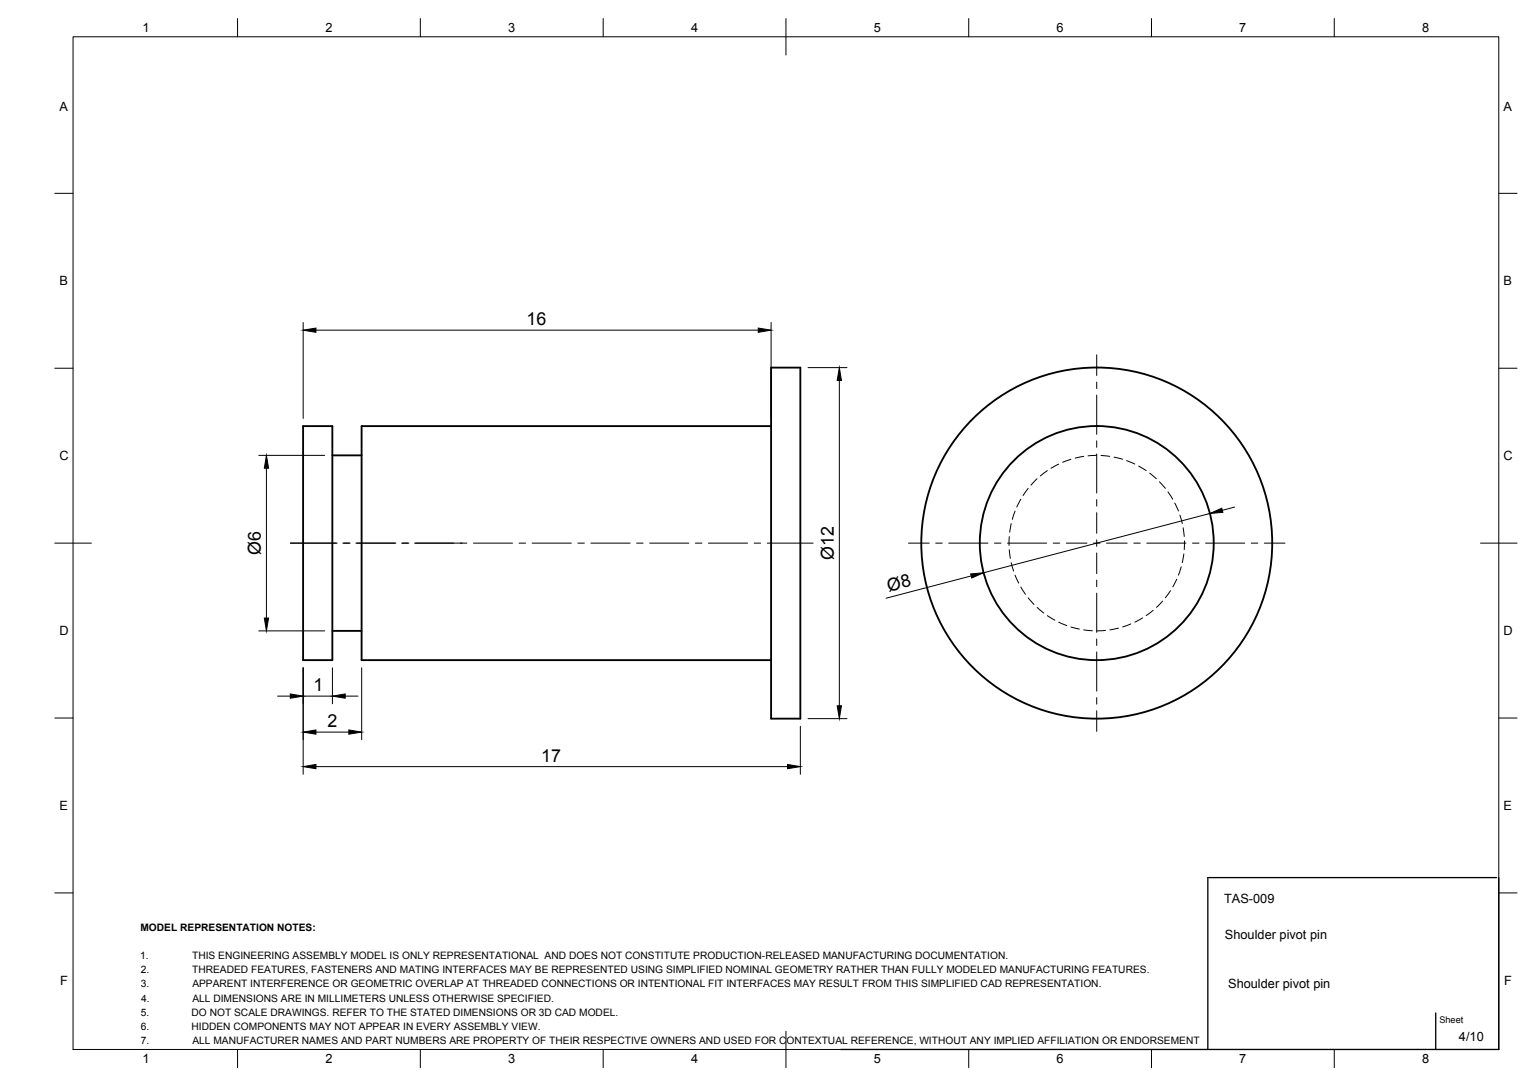
ISO-10303-21;
HEADER;
/* Generated by software containing ST-Developer
 * from STEP Tools, Inc. (www.steptools.com) 
 */

FILE_DESCRIPTION(
/* description */ (''),
/* implementation_level */ '2;1');

FILE_NAME(
/* name */ 'Shoulder pivot pin.step',
/* time_stamp */ '2026-11-12T00:53:40-08:00',
/* author */ (''),
/* organization */ (''),
/* preprocessor_version */ 'ST-DEVELOPER v20.2',
/* originating_system */ 'Autodesk Translation Framework v15.17.0.0',
/* authorisation */ '');

FILE_SCHEMA (('AUTOMOTIVE_DESIGN { 1 0 10303 214 3 1 1 }'));
ENDSEC;

DATA;
#10=MECHANICAL_DESIGN_GEOMETRIC_PRESENTATION_REPRESENTATION('',(#573),#22129);
#555=SHAPE_REPRESENTATION_RELATIONSHIP('SRR','None',#22174,#564);
#564=ADVANCED_BREP_SHAPE_REPRESENTATION('',(#582),#22120);
#573=STYLED_ITEM('',(#22233),#582);
#582=MANIFOLD_SOLID_BREP('Body1',#8804);
#596=FACE_BOUND('',#1528,.T.);
#597=FACE_BOUND('',#1530,.T.);
#598=FACE_BOUND('',#1533,.T.);
#780=PLANE('',#9062);
#781=PLANE('',#9064);
#782=PLANE('',#9068);
#783=PLANE('',#9073);
#784=PLANE('',#9075);
#1037=FACE_OUTER_BOUND('',#1526,.T.);
#1038=FACE_OUTER_BOUND('',#1527,.T.);
#1039=FACE_OUTER_BOUND('',#1529,.T.);
#1040=FACE_OUTER_BOUND('',#1531,.T.);
#1041=FACE_OUTER_BOUND('',#1532,.T.);
#1042=FACE_OUTER_BOUND('',#1534,.T.);
#1043=FACE_OUTER_BOUND('',#1535,.T.);
#1044=FACE_OUTER_BOUND('',#1536,.T.);
#1045=FACE_OUTER_BOUND('',#1537,.T.);
#1526=EDGE_LOOP('',(#6438,#6439,#6440,#6441));
#1527=EDGE_LOOP('',(#6442));
#1528=EDGE_LOOP('',(#6443));
#1529=EDGE_LOOP('',(#6444));
#1530=EDGE_LOOP('',(#6445));
#1531=EDGE_LOOP('',(#6446,#6447,#6448,#6449));
#1532=EDGE_LOOP('',(#6450));
#1533=EDGE_LOOP('',(#6451));
#1534=EDGE_LOOP('',(#6452,#6453,#6454,#6455));
#1535=EDGE_LOOP('',(#6456));
#1536=EDGE_LOOP('',(#6457,#6458,#6459,#6460));
#1537=EDGE_LOOP('',(#6461));
#2316=LINE('',#12207,#3046);
#2317=LINE('',#12218,#3047);
#2318=LINE('',#12226,#3048);
#2319=LINE('',#12230,#3049);
#3046=VECTOR('',#10184,0.3);
#3047=VECTOR('',#10199,0.4);
#3048=VECTOR('',#10208,0.6);
#3049=VECTOR('',#10215,0.4);
#3400=CIRCLE('',#9060,0.3);
#3401=CIRCLE('',#9061,0.3);
#3402=CIRCLE('',#9063,0.4);
#3403=CIRCLE('',#9065,0.4);
#3404=CIRCLE('',#9067,0.4);
#3405=CIRCLE('',#9069,0.6);
#3406=CIRCLE('',#9070,0.4);
#3407=CIRCLE('',#9072,0.6);
#3812=VERTEX_POINT('',#12204);
#3813=VERTEX_POINT('',#12206);
#3814=VERTEX_POINT('',#12210);
#3815=VERTEX_POINT('',#12213);
#3816=VERTEX_POINT('',#12216);
#3817=VERTEX_POINT('',#12220);
#3818=VERTEX_POINT('',#12222);
#3819=VERTEX_POINT('',#12225);
#4772=EDGE_CURVE('',#3812,#3812,#3400,.T.);
#4773=EDGE_CURVE('',#3812,#3813,#2316,.T.);
#4774=EDGE_CURVE('',#3813,#3813,#3401,.T.);
#4775=EDGE_CURVE('',#3814,#3814,#3402,.T.);
#4776=EDGE_CURVE('',#3815,#3815,#3403,.T.);
#4777=EDGE_CURVE('',#3816,#3816,#3404,.T.);
#4778=EDGE_CURVE('',#3816,#3815,#2317,.T.);
#4779=EDGE_CURVE('',#3817,#3817,#3405,.T.);
#4780=EDGE_CURVE('',#3818,#3818,#3406,.T.);
#4781=EDGE_CURVE('',#3817,#3819,#2318,.T.);
#4782=EDGE_CURVE('',#3819,#3819,#3407,.T.);
#4783=EDGE_CURVE('',#3814,#3818,#2319,.T.);
#6438=ORIENTED_EDGE('',*,*,#4772,.T.);
#6439=ORIENTED_EDGE('',*,*,#4773,.T.);
#6440=ORIENTED_EDGE('',*,*,#4774,.F.);
#6441=ORIENTED_EDGE('',*,*,#4773,.F.);
#6442=ORIENTED_EDGE('',*,*,#4775,.F.);
#6443=ORIENTED_EDGE('',*,*,#4772,.F.);
#6444=ORIENTED_EDGE('',*,*,#4776,.F.);
#6445=ORIENTED_EDGE('',*,*,#4774,.T.);
#6446=ORIENTED_EDGE('',*,*,#4777,.F.);
#6447=ORIENTED_EDGE('',*,*,#4778,.T.);
#6448=ORIENTED_EDGE('',*,*,#4776,.T.);
#6449=ORIENTED_EDGE('',*,*,#4778,.F.);
#6450=ORIENTED_EDGE('',*,*,#4779,.T.);
#6451=ORIENTED_EDGE('',*,*,#4780,.F.);
#6452=ORIENTED_EDGE('',*,*,#4779,.F.);
#6453=ORIENTED_EDGE('',*,*,#4781,.T.);
#6454=ORIENTED_EDGE('',*,*,#4782,.T.);
#6455=ORIENTED_EDGE('',*,*,#4781,.F.);
#6456=ORIENTED_EDGE('',*,*,#4782,.F.);
#6457=ORIENTED_EDGE('',*,*,#4775,.T.);
#6458=ORIENTED_EDGE('',*,*,#4783,.T.);
#6459=ORIENTED_EDGE('',*,*,#4780,.T.);
#6460=ORIENTED_EDGE('',*,*,#4783,.F.);
#6461=ORIENTED_EDGE('',*,*,#4777,.T.);
#8191=CYLINDRICAL_SURFACE('',#9059,0.3);
#8192=CYLINDRICAL_SURFACE('',#9066,0.4);
#8193=CYLINDRICAL_SURFACE('',#9071,0.6);
#8194=CYLINDRICAL_SURFACE('',#9074,0.4);
#8454=ADVANCED_FACE('',(#1037),#8191,.T.);
#8455=ADVANCED_FACE('',(#1038,#596),#780,.F.);
#8456=ADVANCED_FACE('',(#1039,#597),#781,.F.);
#8457=ADVANCED_FACE('',(#1040),#8192,.T.);
#8458=ADVANCED_FACE('',(#1041,#598),#782,.T.);
#8459=ADVANCED_FACE('',(#1042),#8193,.T.);
#8460=ADVANCED_FACE('',(#1043),#783,.F.);
#8461=ADVANCED_FACE('',(#1044),#8194,.T.);
#8462=ADVANCED_FACE('',(#1045),#784,.T.);
#8804=CLOSED_SHELL('',(#8454,#8455,#8456,#8457,#8458,#8459,#8460,#8461,
#8462));
#9058=AXIS2_PLACEMENT_3D('',#12202,#10178,#10179);
#9059=AXIS2_PLACEMENT_3D('',#12203,#10180,#10181);
#9060=AXIS2_PLACEMENT_3D('',#12205,#10182,#10183);
#9061=AXIS2_PLACEMENT_3D('',#12208,#10185,#10186);
#9062=AXIS2_PLACEMENT_3D('',#12209,#10187,#10188);
#9063=AXIS2_PLACEMENT_3D('',#12211,#10189,#10190);
#9064=AXIS2_PLACEMENT_3D('',#12212,#10191,#10192);
#9065=AXIS2_PLACEMENT_3D('',#12214,#10193,#10194);
#9066=AXIS2_PLACEMENT_3D('',#12215,#10195,#10196);
#9067=AXIS2_PLACEMENT_3D('',#12217,#10197,#10198);
#9068=AXIS2_PLACEMENT_3D('',#12219,#10200,#10201);
#9069=AXIS2_PLACEMENT_3D('',#12221,#10202,#10203);
#9070=AXIS2_PLACEMENT_3D('',#12223,#10204,#10205);
#9071=AXIS2_PLACEMENT_3D('',#12224,#10206,#10207);
#9072=AXIS2_PLACEMENT_3D('',#12227,#10209,#10210);
#9073=AXIS2_PLACEMENT_3D('',#12228,#10211,#10212);
#9074=AXIS2_PLACEMENT_3D('',#12229,#10213,#10214);
#9075=AXIS2_PLACEMENT_3D('',#12231,#10216,#10217);
#10178=DIRECTION('axis',(0.,0.,1.));
#10179=DIRECTION('refdir',(1.,0.,0.));
#10180=DIRECTION('center_axis',(0.,0.,1.));
#10181=DIRECTION('ref_axis',(1.,0.,0.));
#10182=DIRECTION('center_axis',(0.,0.,1.));
#10183=DIRECTION('ref_axis',(1.,0.,0.));
#10184=DIRECTION('',(0.,0.,1.));
#10185=DIRECTION('center_axis',(0.,0.,1.));
#10186=DIRECTION('ref_axis',(1.,0.,0.));
#10187=DIRECTION('center_axis',(0.,0.,-1.));
#10188=DIRECTION('ref_axis',(-1.,0.,0.));
#10189=DIRECTION('center_axis',(0.,0.,-1.));
#10190=DIRECTION('ref_axis',(1.,0.,0.));
#10191=DIRECTION('center_axis',(0.,0.,1.));
#10192=DIRECTION('ref_axis',(1.,0.,0.));
#10193=DIRECTION('center_axis',(0.,0.,1.));
#10194=DIRECTION('ref_axis',(1.,0.,0.));
#10195=DIRECTION('center_axis',(0.,0.,1.));
#10196=DIRECTION('ref_axis',(1.,0.,0.));
#10197=DIRECTION('center_axis',(0.,0.,1.));
#10198=DIRECTION('ref_axis',(1.,0.,0.));
#10199=DIRECTION('',(0.,0.,-1.));
#10200=DIRECTION('center_axis',(0.,0.,1.));
#10201=DIRECTION('ref_axis',(1.,0.,0.));
#10202=DIRECTION('center_axis',(0.,0.,1.));
#10203=DIRECTION('ref_axis',(1.,0.,0.));
#10204=DIRECTION('center_axis',(0.,0.,1.));
#10205=DIRECTION('ref_axis',(1.,0.,0.));
#10206=DIRECTION('center_axis',(0.,0.,1.));
#10207=DIRECTION('ref_axis',(1.,0.,0.));
#10208=DIRECTION('',(0.,0.,-1.));
#10209=DIRECTION('center_axis',(0.,0.,1.));
#10210=DIRECTION('ref_axis',(1.,0.,0.));
#10211=DIRECTION('center_axis',(0.,0.,1.));
#10212=DIRECTION('ref_axis',(1.,0.,0.));
#10213=DIRECTION('center_axis',(0.,0.,1.));
#10214=DIRECTION('ref_axis',(1.,0.,0.));
#10215=DIRECTION('',(0.,0.,-1.));
#10216=DIRECTION('center_axis',(0.,0.,1.));
#10217=DIRECTION('ref_axis',(1.,0.,0.));
#12202=CARTESIAN_POINT('',(0.,0.,0.));
#12203=CARTESIAN_POINT('Origin',(0.,0.,0.75));
#12204=CARTESIAN_POINT('',(-0.3,-3.67394039744206E-17,0.7));
#12205=CARTESIAN_POINT('Origin',(0.,0.,0.7));
#12206=CARTESIAN_POINT('',(-0.3,-3.67394039744206E-17,0.8));
#12207=CARTESIAN_POINT('',(-0.3,-3.67394039744206E-17,0.75));
#12208=CARTESIAN_POINT('Origin',(0.,0.,0.8));
#12209=CARTESIAN_POINT('Origin',(0.7,0.,0.7));
#12210=CARTESIAN_POINT('',(-0.4,4.89858719658941E-17,0.7));
#12211=CARTESIAN_POINT('Origin',(0.,0.,0.7));
#12212=CARTESIAN_POINT('Origin',(0.3,0.,0.8));
#12213=CARTESIAN_POINT('',(-0.4,-4.89858719658941E-17,0.8));
#12214=CARTESIAN_POINT('Origin',(0.,0.,0.8));
#12215=CARTESIAN_POINT('Origin',(0.,0.,-0.7));
#12216=CARTESIAN_POINT('',(-0.4,-4.89858719658941E-17,0.9));
#12217=CARTESIAN_POINT('Origin',(0.,0.,0.9));
#12218=CARTESIAN_POINT('',(-0.4,-4.89858719658941E-17,-0.7));
#12219=CARTESIAN_POINT('Origin',(0.,0.,-0.7));
#12220=CARTESIAN_POINT('',(-0.6,-7.34788079488412E-17,-0.7));
#12221=CARTESIAN_POINT('Origin',(0.,0.,-0.7));
#12222=CARTESIAN_POINT('',(-0.4,-4.89858719658941E-17,-0.7));
#12223=CARTESIAN_POINT('Origin',(0.,0.,-0.7));
#12224=CARTESIAN_POINT('Origin',(0.,0.,-0.8));
#12225=CARTESIAN_POINT('',(-0.6,-7.34788079488412E-17,-0.8));
#12226=CARTESIAN_POINT('',(-0.6,-7.34788079488412E-17,-0.8));
#12227=CARTESIAN_POINT('Origin',(0.,0.,-0.8));
#12228=CARTESIAN_POINT('Origin',(0.,0.,-0.8));
#12229=CARTESIAN_POINT('Origin',(0.,0.,-0.7));
#12230=CARTESIAN_POINT('',(-0.4,-4.89858719658941E-17,-0.7));
#12231=CARTESIAN_POINT('Origin',(0.,0.,0.9));
#22108=UNCERTAINTY_MEASURE_WITH_UNIT(LENGTH_MEASURE(0.001),#22130,
'DISTANCE_ACCURACY_VALUE',
'Maximum model space distance between geometric entities at asserted c
onnectivities');
#22117=UNCERTAINTY_MEASURE_WITH_UNIT(LENGTH_MEASURE(0.001),#22130,
'DISTANCE_ACCURACY_VALUE',
'Maximum model space distance between geometric entities at asserted c
onnectivities');
#22120=(
GEOMETRIC_REPRESENTATION_CONTEXT(3)
GLOBAL_UNCERTAINTY_ASSIGNED_CONTEXT((#22108))
GLOBAL_UNIT_ASSIGNED_CONTEXT((#22130,#22132,#22133))
REPRESENTATION_CONTEXT('','3D')
);
#22129=(
GEOMETRIC_REPRESENTATION_CONTEXT(3)
GLOBAL_UNCERTAINTY_ASSIGNED_CONTEXT((#22117))
GLOBAL_UNIT_ASSIGNED_CONTEXT((#22130,#22132,#22133))
REPRESENTATION_CONTEXT('','3D')
);
#22130=(
LENGTH_UNIT()
NAMED_UNIT(*)
SI_UNIT(.CENTI.,.METRE.)
);
#22132=(
NAMED_UNIT(*)
PLANE_ANGLE_UNIT()
SI_UNIT($,.RADIAN.)
);
#22133=(
NAMED_UNIT(*)
SI_UNIT($,.STERADIAN.)
SOLID_ANGLE_UNIT()
);
#22136=SHAPE_DEFINITION_REPRESENTATION(#22147,#22174);
#22147=PRODUCT_DEFINITION_SHAPE('',$,#22186);
#22174=SHAPE_REPRESENTATION('',(#9058),#22120);
#22183=PRODUCT_DEFINITION_CONTEXT('part definition',#22218,'design');
#22186=PRODUCT_DEFINITION('Shoulder pivot pin','Shoulder pivot pin',#22197,
#22183);
#22197=PRODUCT_DEFINITION_FORMATION('',$,#22222);
#22218=APPLICATION_CONTEXT(
'Core Data for Automotive Mechanical Design Process');
#22219=PRODUCT_CONTEXT('part definition',#22218,'mechanical');
#22222=PRODUCT('Shoulder pivot pin','Shoulder pivot pin',$,(#22219));
#22233=PRESENTATION_STYLE_ASSIGNMENT((#22241));
#22241=SURFACE_STYLE_USAGE(.BOTH.,#22249);
#22249=SURFACE_SIDE_STYLE('',(#22257));
#22257=SURFACE_STYLE_FILL_AREA(#22265);
#22265=FILL_AREA_STYLE('Pivot dark gray',(#22273));
#22273=FILL_AREA_STYLE_COLOUR('Pivot dark gray',#22281);
#22281=COLOUR_RGB('Pivot dark gray',0.27843137254902,0.309803921568627,
0.352941176470588);
ENDSEC;
END-ISO-10303-21;
